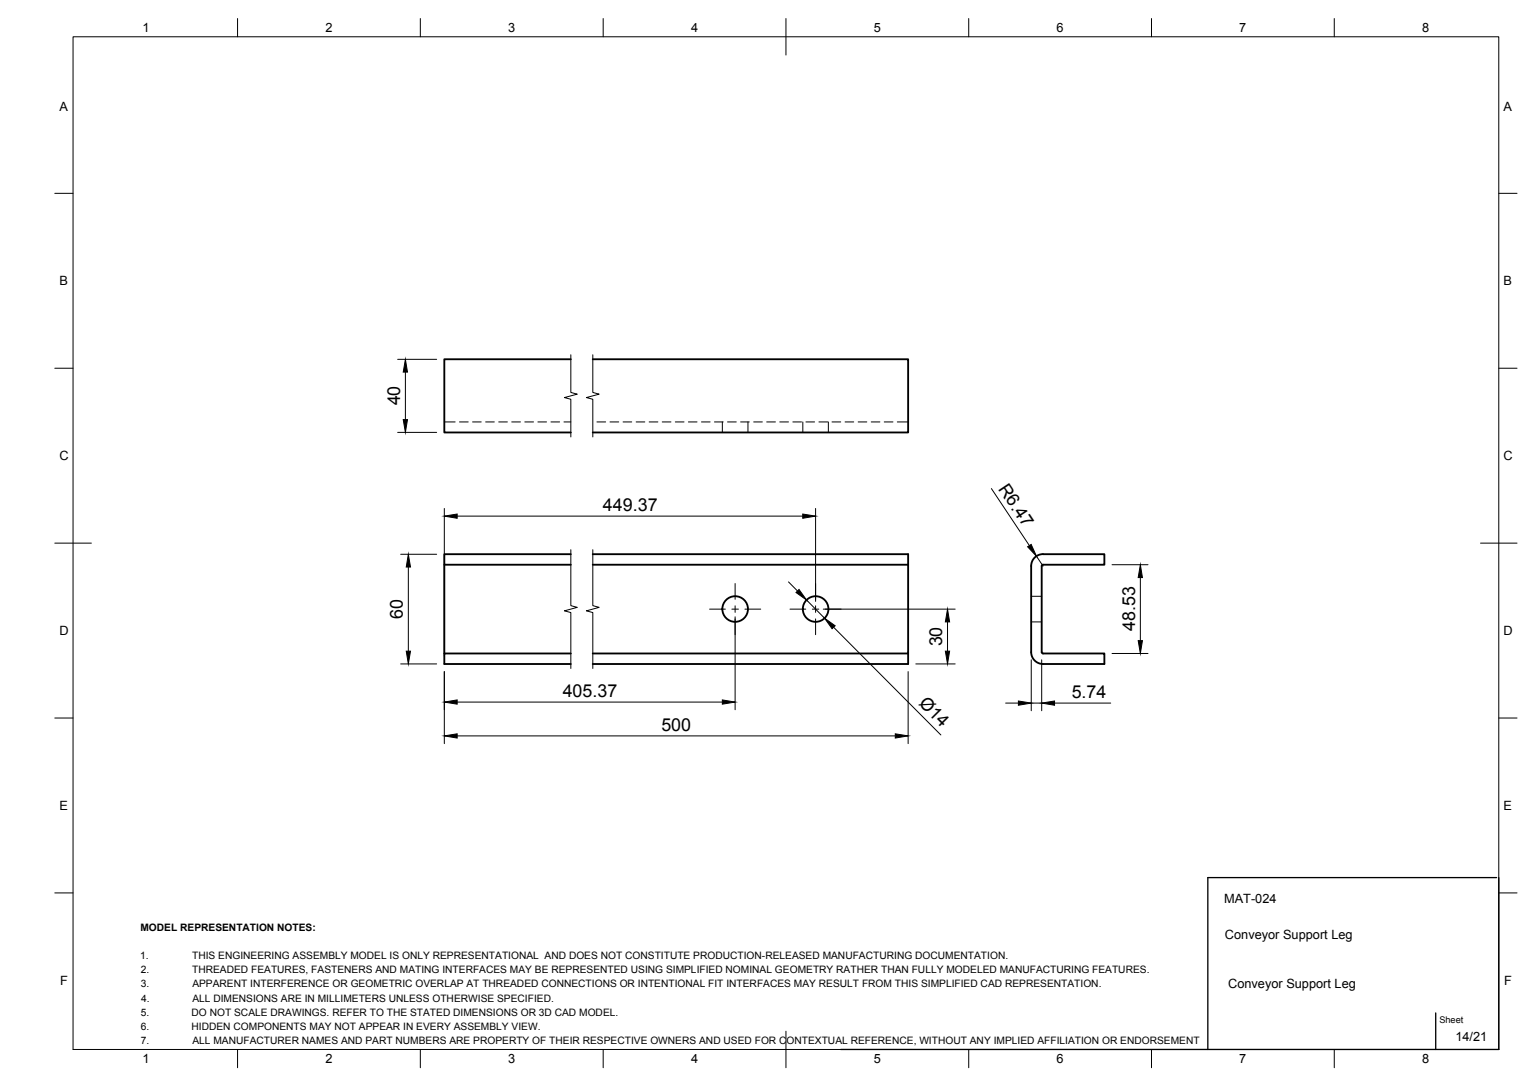
ISO-10303-21;
HEADER;
/* Generated by software containing ST-Developer
 * from STEP Tools, Inc. (www.steptools.com) 
 */

FILE_DESCRIPTION(
/* description */ ('STEP AP214'),
/* implementation_level */ '2;1');

FILE_NAME(
/* name */ 'Conveyor Support Leg.step',
/* time_stamp */ '2026-11-14T06:34:07-08:00',
/* author */ (''),
/* organization */ (''),
/* preprocessor_version */ 'ST-DEVELOPER v20.2',
/* originating_system */ 'Autodesk Translation Framework v15.17.0.0',
/* authorisation */ '');

FILE_SCHEMA (('AUTOMOTIVE_DESIGN { 1 0 10303 214 3 1 1 }'));
ENDSEC;

DATA;
#10=MECHANICAL_DESIGN_GEOMETRIC_PRESENTATION_REPRESENTATION('',(#7321),#310623);
#7236=SHAPE_REPRESENTATION_RELATIONSHIP('SRR','None',#310910,#7253);
#7253=ADVANCED_BREP_SHAPE_REPRESENTATION('',(#7388),#310619);
#7321=STYLED_ITEM('',(#311003),#7388);
#7388=MANIFOLD_SOLID_BREP('Body1',#93772);
#7692=FACE_BOUND('',#20319,.T.);
#7693=FACE_BOUND('',#20320,.T.);
#7694=FACE_BOUND('',#20324,.T.);
#7695=FACE_BOUND('',#20325,.T.);
#8642=PLANE('',#104604);
#8643=PLANE('',#104605);
#8644=PLANE('',#104606);
#8645=PLANE('',#104607);
#8646=PLANE('',#104608);
#8647=PLANE('',#104609);
#8648=PLANE('',#104610);
#8649=PLANE('',#104611);
#8650=PLANE('',#104612);
#8651=PLANE('',#104615);
#8652=PLANE('',#104616);
#8653=PLANE('',#104619);
#8654=PLANE('',#104622);
#8655=PLANE('',#104625);
#8656=PLANE('',#104627);
#8657=PLANE('',#104630);
#8658=PLANE('',#104632);
#8659=PLANE('',#104633);
#14261=FACE_OUTER_BOUND('',#20301,.T.);
#14262=FACE_OUTER_BOUND('',#20302,.T.);
#14263=FACE_OUTER_BOUND('',#20303,.T.);
#14264=FACE_OUTER_BOUND('',#20304,.T.);
#14265=FACE_OUTER_BOUND('',#20305,.T.);
#14266=FACE_OUTER_BOUND('',#20306,.T.);
#14267=FACE_OUTER_BOUND('',#20307,.T.);
#14268=FACE_OUTER_BOUND('',#20308,.T.);
#14269=FACE_OUTER_BOUND('',#20309,.T.);
#14270=FACE_OUTER_BOUND('',#20310,.T.);
#14271=FACE_OUTER_BOUND('',#20311,.T.);
#14272=FACE_OUTER_BOUND('',#20312,.T.);
#14273=FACE_OUTER_BOUND('',#20313,.T.);
#14274=FACE_OUTER_BOUND('',#20314,.T.);
#14275=FACE_OUTER_BOUND('',#20315,.T.);
#14276=FACE_OUTER_BOUND('',#20316,.T.);
#14277=FACE_OUTER_BOUND('',#20317,.T.);
#14278=FACE_OUTER_BOUND('',#20318,.T.);
#14279=FACE_OUTER_BOUND('',#20321,.T.);
#14280=FACE_OUTER_BOUND('',#20322,.T.);
#14281=FACE_OUTER_BOUND('',#20323,.T.);
#14282=FACE_OUTER_BOUND('',#20326,.T.);
#14283=FACE_OUTER_BOUND('',#20327,.T.);
#14284=FACE_OUTER_BOUND('',#20328,.T.);
#20301=EDGE_LOOP('',(#84911,#84912,#84913,#84914));
#20302=EDGE_LOOP('',(#84915,#84916,#84917,#84918));
#20303=EDGE_LOOP('',(#84919,#84920,#84921,#84922));
#20304=EDGE_LOOP('',(#84923,#84924,#84925,#84926));
#20305=EDGE_LOOP('',(#84927,#84928,#84929,#84930));
#20306=EDGE_LOOP('',(#84931,#84932,#84933,#84934));
#20307=EDGE_LOOP('',(#84935,#84936,#84937,#84938));
#20308=EDGE_LOOP('',(#84939,#84940,#84941,#84942));
#20309=EDGE_LOOP('',(#84943,#84944,#84945,#84946));
#20310=EDGE_LOOP('',(#84947,#84948,#84949,#84950));
#20311=EDGE_LOOP('',(#84951,#84952,#84953,#84954));
#20312=EDGE_LOOP('',(#84955,#84956,#84957,#84958));
#20313=EDGE_LOOP('',(#84959,#84960,#84961,#84962));
#20314=EDGE_LOOP('',(#84963,#84964,#84965,#84966));
#20315=EDGE_LOOP('',(#84967,#84968,#84969,#84970));
#20316=EDGE_LOOP('',(#84971,#84972,#84973,#84974));
#20317=EDGE_LOOP('',(#84975,#84976,#84977,#84978));
#20318=EDGE_LOOP('',(#84979,#84980,#84981,#84982));
#20319=EDGE_LOOP('',(#84983));
#20320=EDGE_LOOP('',(#84984));
#20321=EDGE_LOOP('',(#84985,#84986,#84987,#84988));
#20322=EDGE_LOOP('',(#84989,#84990,#84991,#84992));
#20323=EDGE_LOOP('',(#84993,#84994,#84995,#84996));
#20324=EDGE_LOOP('',(#84997));
#20325=EDGE_LOOP('',(#84998));
#20326=EDGE_LOOP('',(#84999,#85000,#85001,#85002));
#20327=EDGE_LOOP('',(#85003,#85004,#85005,#85006));
#20328=EDGE_LOOP('',(#85007,#85008,#85009,#85010));
#24672=LINE('',#302915,#29019);
#24673=LINE('',#302921,#29020);
#24674=LINE('',#302926,#29021);
#24675=LINE('',#302928,#29022);
#24676=LINE('',#302930,#29023);
#24677=LINE('',#302931,#29024);
#24678=LINE('',#302935,#29025);
#24679=LINE('',#302937,#29026);
#24680=LINE('',#302939,#29027);
#24681=LINE('',#302940,#29028);
#24682=LINE('',#302943,#29029);
#24683=LINE('',#302945,#29030);
#24684=LINE('',#302946,#29031);
#24685=LINE('',#302949,#29032);
#24686=LINE('',#302951,#29033);
#24687=LINE('',#302952,#29034);
#24688=LINE('',#302955,#29035);
#24689=LINE('',#302957,#29036);
#24690=LINE('',#302958,#29037);
#24691=LINE('',#302961,#29038);
#24692=LINE('',#302963,#29039);
#24693=LINE('',#302964,#29040);
#24694=LINE('',#302966,#29041);
#24695=LINE('',#302967,#29042);
#24696=LINE('',#302969,#29043);
#24697=LINE('',#302970,#29044);
#24698=LINE('',#302974,#29045);
#24699=LINE('',#302979,#29046);
#24700=LINE('',#302981,#29047);
#24701=LINE('',#302982,#29048);
#24702=LINE('',#302987,#29049);
#24703=LINE('',#302995,#29050);
#24704=LINE('',#302999,#29051);
#24705=LINE('',#303000,#29052);
#24706=LINE('',#303002,#29053);
#24707=LINE('',#303004,#29054);
#24708=LINE('',#303007,#29055);
#24709=LINE('',#303009,#29056);
#29019=VECTOR('',#130329,7.00000000000001);
#29020=VECTOR('',#130336,7.);
#29021=VECTOR('',#130341,1000.);
#29022=VECTOR('',#130342,1000.);
#29023=VECTOR('',#130343,1000.);
#29024=VECTOR('',#130344,1000.);
#29025=VECTOR('',#130347,1000.);
#29026=VECTOR('',#130348,1000.);
#29027=VECTOR('',#130349,1000.);
#29028=VECTOR('',#130350,1000.);
#29029=VECTOR('',#130353,1000.);
#29030=VECTOR('',#130354,1000.);
#29031=VECTOR('',#130355,1000.);
#29032=VECTOR('',#130358,1000.);
#29033=VECTOR('',#130359,1000.);
#29034=VECTOR('',#130360,1000.);
#29035=VECTOR('',#130363,1000.);
#29036=VECTOR('',#130364,1000.);
#29037=VECTOR('',#130365,1000.);
#29038=VECTOR('',#130368,1000.);
#29039=VECTOR('',#130369,1000.);
#29040=VECTOR('',#130370,1000.);
#29041=VECTOR('',#130373,1000.);
#29042=VECTOR('',#130374,1000.);
#29043=VECTOR('',#130377,1000.);
#29044=VECTOR('',#130378,1000.);
#29045=VECTOR('',#130381,1000.);
#29046=VECTOR('',#130388,1000.);
#29047=VECTOR('',#130389,1000.);
#29048=VECTOR('',#130390,1000.);
#29049=VECTOR('',#130395,1000.);
#29050=VECTOR('',#130406,1000.);
#29051=VECTOR('',#130413,1000.);
#29052=VECTOR('',#130414,1000.);
#29053=VECTOR('',#130417,1000.);
#29054=VECTOR('',#130420,1000.);
#29055=VECTOR('',#130425,1000.);
#29056=VECTOR('',#130428,1000.);
#35057=CIRCLE('',#104599,7.00000000000001);
#35058=CIRCLE('',#104600,7.00000000000001);
#35059=CIRCLE('',#104602,7.);
#35060=CIRCLE('',#104603,7.);
#35061=CIRCLE('',#104613,6.4732);
#35062=CIRCLE('',#104614,0.736599999999997);
#35063=CIRCLE('',#104617,6.4732);
#35064=CIRCLE('',#104618,0.736599999999997);
#35065=CIRCLE('',#104620,6.4732);
#35066=CIRCLE('',#104621,0.736599999999997);
#35067=CIRCLE('',#104623,6.4732);
#35068=CIRCLE('',#104624,0.736599999999997);
#43338=VERTEX_POINT('',#302912);
#43339=VERTEX_POINT('',#302914);
#43340=VERTEX_POINT('',#302918);
#43341=VERTEX_POINT('',#302920);
#43342=VERTEX_POINT('',#302924);
#43343=VERTEX_POINT('',#302925);
#43344=VERTEX_POINT('',#302927);
#43345=VERTEX_POINT('',#302929);
#43346=VERTEX_POINT('',#302933);
#43347=VERTEX_POINT('',#302934);
#43348=VERTEX_POINT('',#302936);
#43349=VERTEX_POINT('',#302938);
#43350=VERTEX_POINT('',#302942);
#43351=VERTEX_POINT('',#302944);
#43352=VERTEX_POINT('',#302948);
#43353=VERTEX_POINT('',#302950);
#43354=VERTEX_POINT('',#302954);
#43355=VERTEX_POINT('',#302956);
#43356=VERTEX_POINT('',#302960);
#43357=VERTEX_POINT('',#302962);
#43358=VERTEX_POINT('',#302972);
#43359=VERTEX_POINT('',#302973);
#43360=VERTEX_POINT('',#302978);
#43361=VERTEX_POINT('',#302980);
#43362=VERTEX_POINT('',#302984);
#43363=VERTEX_POINT('',#302986);
#43364=VERTEX_POINT('',#302993);
#43365=VERTEX_POINT('',#302994);
#57235=EDGE_CURVE('',#43338,#43338,#35057,.T.);
#57236=EDGE_CURVE('',#43338,#43339,#24672,.T.);
#57237=EDGE_CURVE('',#43339,#43339,#35058,.T.);
#57238=EDGE_CURVE('',#43340,#43340,#35059,.T.);
#57239=EDGE_CURVE('',#43340,#43341,#24673,.T.);
#57240=EDGE_CURVE('',#43341,#43341,#35060,.T.);
#57241=EDGE_CURVE('',#43342,#43343,#24674,.T.);
#57242=EDGE_CURVE('',#43342,#43344,#24675,.T.);
#57243=EDGE_CURVE('',#43344,#43345,#24676,.T.);
#57244=EDGE_CURVE('',#43345,#43343,#24677,.T.);
#57245=EDGE_CURVE('',#43346,#43347,#24678,.T.);
#57246=EDGE_CURVE('',#43347,#43348,#24679,.T.);
#57247=EDGE_CURVE('',#43349,#43348,#24680,.T.);
#57248=EDGE_CURVE('',#43349,#43346,#24681,.T.);
#57249=EDGE_CURVE('',#43347,#43350,#24682,.T.);
#57250=EDGE_CURVE('',#43346,#43351,#24683,.T.);
#57251=EDGE_CURVE('',#43351,#43350,#24684,.T.);
#57252=EDGE_CURVE('',#43348,#43352,#24685,.T.);
#57253=EDGE_CURVE('',#43353,#43352,#24686,.T.);
#57254=EDGE_CURVE('',#43349,#43353,#24687,.T.);
#57255=EDGE_CURVE('',#43344,#43354,#24688,.T.);
#57256=EDGE_CURVE('',#43354,#43355,#24689,.T.);
#57257=EDGE_CURVE('',#43355,#43345,#24690,.T.);
#57258=EDGE_CURVE('',#43342,#43356,#24691,.T.);
#57259=EDGE_CURVE('',#43357,#43343,#24692,.T.);
#57260=EDGE_CURVE('',#43356,#43357,#24693,.T.);
#57261=EDGE_CURVE('',#43354,#43356,#24694,.T.);
#57262=EDGE_CURVE('',#43357,#43355,#24695,.T.);
#57263=EDGE_CURVE('',#43350,#43352,#24696,.T.);
#57264=EDGE_CURVE('',#43351,#43353,#24697,.T.);
#57265=EDGE_CURVE('',#43358,#43359,#24698,.T.);
#57266=EDGE_CURVE('',#43355,#43358,#35061,.T.);
#57267=EDGE_CURVE('',#43357,#43359,#35062,.T.);
#57268=EDGE_CURVE('',#43358,#43360,#24699,.T.);
#57269=EDGE_CURVE('',#43359,#43361,#24700,.T.);
#57270=EDGE_CURVE('',#43361,#43360,#24701,.T.);
#57271=EDGE_CURVE('',#43345,#43362,#35063,.T.);
#57272=EDGE_CURVE('',#43363,#43362,#24702,.T.);
#57273=EDGE_CURVE('',#43343,#43363,#35064,.T.);
#57274=EDGE_CURVE('',#43360,#43349,#35065,.T.);
#57275=EDGE_CURVE('',#43361,#43346,#35066,.T.);
#57276=EDGE_CURVE('',#43364,#43365,#24703,.T.);
#57277=EDGE_CURVE('',#43364,#43353,#35067,.T.);
#57278=EDGE_CURVE('',#43365,#43351,#35068,.T.);
#57279=EDGE_CURVE('',#43362,#43364,#24704,.T.);
#57280=EDGE_CURVE('',#43363,#43365,#24705,.T.);
#57281=EDGE_CURVE('',#43360,#43364,#24706,.T.);
#57282=EDGE_CURVE('',#43358,#43362,#24707,.T.);
#57283=EDGE_CURVE('',#43359,#43363,#24708,.T.);
#57284=EDGE_CURVE('',#43361,#43365,#24709,.T.);
#84911=ORIENTED_EDGE('',*,*,#57235,.F.);
#84912=ORIENTED_EDGE('',*,*,#57236,.T.);
#84913=ORIENTED_EDGE('',*,*,#57237,.T.);
#84914=ORIENTED_EDGE('',*,*,#57236,.F.);
#84915=ORIENTED_EDGE('',*,*,#57238,.F.);
#84916=ORIENTED_EDGE('',*,*,#57239,.T.);
#84917=ORIENTED_EDGE('',*,*,#57240,.T.);
#84918=ORIENTED_EDGE('',*,*,#57239,.F.);
#84919=ORIENTED_EDGE('',*,*,#57241,.F.);
#84920=ORIENTED_EDGE('',*,*,#57242,.T.);
#84921=ORIENTED_EDGE('',*,*,#57243,.T.);
#84922=ORIENTED_EDGE('',*,*,#57244,.T.);
#84923=ORIENTED_EDGE('',*,*,#57245,.T.);
#84924=ORIENTED_EDGE('',*,*,#57246,.T.);
#84925=ORIENTED_EDGE('',*,*,#57247,.F.);
#84926=ORIENTED_EDGE('',*,*,#57248,.T.);
#84927=ORIENTED_EDGE('',*,*,#57249,.F.);
#84928=ORIENTED_EDGE('',*,*,#57245,.F.);
#84929=ORIENTED_EDGE('',*,*,#57250,.T.);
#84930=ORIENTED_EDGE('',*,*,#57251,.T.);
#84931=ORIENTED_EDGE('',*,*,#57247,.T.);
#84932=ORIENTED_EDGE('',*,*,#57252,.T.);
#84933=ORIENTED_EDGE('',*,*,#57253,.F.);
#84934=ORIENTED_EDGE('',*,*,#57254,.F.);
#84935=ORIENTED_EDGE('',*,*,#57243,.F.);
#84936=ORIENTED_EDGE('',*,*,#57255,.T.);
#84937=ORIENTED_EDGE('',*,*,#57256,.T.);
#84938=ORIENTED_EDGE('',*,*,#57257,.T.);
#84939=ORIENTED_EDGE('',*,*,#57258,.F.);
#84940=ORIENTED_EDGE('',*,*,#57241,.T.);
#84941=ORIENTED_EDGE('',*,*,#57259,.F.);
#84942=ORIENTED_EDGE('',*,*,#57260,.F.);
#84943=ORIENTED_EDGE('',*,*,#57256,.F.);
#84944=ORIENTED_EDGE('',*,*,#57261,.T.);
#84945=ORIENTED_EDGE('',*,*,#57260,.T.);
#84946=ORIENTED_EDGE('',*,*,#57262,.T.);
#84947=ORIENTED_EDGE('',*,*,#57263,.F.);
#84948=ORIENTED_EDGE('',*,*,#57251,.F.);
#84949=ORIENTED_EDGE('',*,*,#57264,.T.);
#84950=ORIENTED_EDGE('',*,*,#57253,.T.);
#84951=ORIENTED_EDGE('',*,*,#57265,.F.);
#84952=ORIENTED_EDGE('',*,*,#57266,.F.);
#84953=ORIENTED_EDGE('',*,*,#57262,.F.);
#84954=ORIENTED_EDGE('',*,*,#57267,.T.);
#84955=ORIENTED_EDGE('',*,*,#57268,.F.);
#84956=ORIENTED_EDGE('',*,*,#57265,.T.);
#84957=ORIENTED_EDGE('',*,*,#57269,.T.);
#84958=ORIENTED_EDGE('',*,*,#57270,.T.);
#84959=ORIENTED_EDGE('',*,*,#57244,.F.);
#84960=ORIENTED_EDGE('',*,*,#57271,.T.);
#84961=ORIENTED_EDGE('',*,*,#57272,.F.);
#84962=ORIENTED_EDGE('',*,*,#57273,.F.);
#84963=ORIENTED_EDGE('',*,*,#57248,.F.);
#84964=ORIENTED_EDGE('',*,*,#57274,.F.);
#84965=ORIENTED_EDGE('',*,*,#57270,.F.);
#84966=ORIENTED_EDGE('',*,*,#57275,.T.);
#84967=ORIENTED_EDGE('',*,*,#57276,.F.);
#84968=ORIENTED_EDGE('',*,*,#57277,.T.);
#84969=ORIENTED_EDGE('',*,*,#57264,.F.);
#84970=ORIENTED_EDGE('',*,*,#57278,.F.);
#84971=ORIENTED_EDGE('',*,*,#57279,.T.);
#84972=ORIENTED_EDGE('',*,*,#57276,.T.);
#84973=ORIENTED_EDGE('',*,*,#57280,.F.);
#84974=ORIENTED_EDGE('',*,*,#57272,.T.);
#84975=ORIENTED_EDGE('',*,*,#57277,.F.);
#84976=ORIENTED_EDGE('',*,*,#57281,.F.);
#84977=ORIENTED_EDGE('',*,*,#57274,.T.);
#84978=ORIENTED_EDGE('',*,*,#57254,.T.);
#84979=ORIENTED_EDGE('',*,*,#57279,.F.);
#84980=ORIENTED_EDGE('',*,*,#57282,.F.);
#84981=ORIENTED_EDGE('',*,*,#57268,.T.);
#84982=ORIENTED_EDGE('',*,*,#57281,.T.);
#84983=ORIENTED_EDGE('',*,*,#57237,.F.);
#84984=ORIENTED_EDGE('',*,*,#57240,.F.);
#84985=ORIENTED_EDGE('',*,*,#57271,.F.);
#84986=ORIENTED_EDGE('',*,*,#57257,.F.);
#84987=ORIENTED_EDGE('',*,*,#57266,.T.);
#84988=ORIENTED_EDGE('',*,*,#57282,.T.);
#84989=ORIENTED_EDGE('',*,*,#57273,.T.);
#84990=ORIENTED_EDGE('',*,*,#57283,.F.);
#84991=ORIENTED_EDGE('',*,*,#57267,.F.);
#84992=ORIENTED_EDGE('',*,*,#57259,.T.);
#84993=ORIENTED_EDGE('',*,*,#57280,.T.);
#84994=ORIENTED_EDGE('',*,*,#57284,.F.);
#84995=ORIENTED_EDGE('',*,*,#57269,.F.);
#84996=ORIENTED_EDGE('',*,*,#57283,.T.);
#84997=ORIENTED_EDGE('',*,*,#57235,.T.);
#84998=ORIENTED_EDGE('',*,*,#57238,.T.);
#84999=ORIENTED_EDGE('',*,*,#57278,.T.);
#85000=ORIENTED_EDGE('',*,*,#57250,.F.);
#85001=ORIENTED_EDGE('',*,*,#57275,.F.);
#85002=ORIENTED_EDGE('',*,*,#57284,.T.);
#85003=ORIENTED_EDGE('',*,*,#57249,.T.);
#85004=ORIENTED_EDGE('',*,*,#57263,.T.);
#85005=ORIENTED_EDGE('',*,*,#57252,.F.);
#85006=ORIENTED_EDGE('',*,*,#57246,.F.);
#85007=ORIENTED_EDGE('',*,*,#57258,.T.);
#85008=ORIENTED_EDGE('',*,*,#57261,.F.);
#85009=ORIENTED_EDGE('',*,*,#57255,.F.);
#85010=ORIENTED_EDGE('',*,*,#57242,.F.);
#87908=CYLINDRICAL_SURFACE('',#104598,7.00000000000001);
#87909=CYLINDRICAL_SURFACE('',#104601,7.);
#87910=CYLINDRICAL_SURFACE('',#104626,6.4732);
#87911=CYLINDRICAL_SURFACE('',#104628,6.4732);
#87912=CYLINDRICAL_SURFACE('',#104629,0.7366);
#87913=CYLINDRICAL_SURFACE('',#104631,0.736599999999997);
#93540=ADVANCED_FACE('',(#14261),#87908,.F.);
#93541=ADVANCED_FACE('',(#14262),#87909,.F.);
#93542=ADVANCED_FACE('',(#14263),#8642,.T.);
#93543=ADVANCED_FACE('',(#14264),#8643,.T.);
#93544=ADVANCED_FACE('',(#14265),#8644,.F.);
#93545=ADVANCED_FACE('',(#14266),#8645,.T.);
#93546=ADVANCED_FACE('',(#14267),#8646,.T.);
#93547=ADVANCED_FACE('',(#14268),#8647,.F.);
#93548=ADVANCED_FACE('',(#14269),#8648,.T.);
#93549=ADVANCED_FACE('',(#14270),#8649,.F.);
#93550=ADVANCED_FACE('',(#14271),#8650,.T.);
#93551=ADVANCED_FACE('',(#14272),#8651,.T.);
#93552=ADVANCED_FACE('',(#14273),#8652,.T.);
#93553=ADVANCED_FACE('',(#14274),#8653,.T.);
#93554=ADVANCED_FACE('',(#14275),#8654,.T.);
#93555=ADVANCED_FACE('',(#14276),#8655,.T.);
#93556=ADVANCED_FACE('',(#14277),#87910,.T.);
#93557=ADVANCED_FACE('',(#14278,#7692,#7693),#8656,.T.);
#93558=ADVANCED_FACE('',(#14279),#87911,.T.);
#93559=ADVANCED_FACE('',(#14280),#87912,.F.);
#93560=ADVANCED_FACE('',(#14281,#7694,#7695),#8657,.F.);
#93561=ADVANCED_FACE('',(#14282),#87913,.F.);
#93562=ADVANCED_FACE('',(#14283),#8658,.T.);
#93563=ADVANCED_FACE('',(#14284),#8659,.T.);
#93772=CLOSED_SHELL('',(#93540,#93541,#93542,#93543,#93544,#93545,#93546,
#93547,#93548,#93549,#93550,#93551,#93552,#93553,#93554,#93555,#93556,#93557,
#93558,#93559,#93560,#93561,#93562,#93563));
#104597=AXIS2_PLACEMENT_3D('',#302910,#130323,#130324);
#104598=AXIS2_PLACEMENT_3D('',#302911,#130325,#130326);
#104599=AXIS2_PLACEMENT_3D('',#302913,#130327,#130328);
#104600=AXIS2_PLACEMENT_3D('',#302916,#130330,#130331);
#104601=AXIS2_PLACEMENT_3D('',#302917,#130332,#130333);
#104602=AXIS2_PLACEMENT_3D('',#302919,#130334,#130335);
#104603=AXIS2_PLACEMENT_3D('',#302922,#130337,#130338);
#104604=AXIS2_PLACEMENT_3D('',#302923,#130339,#130340);
#104605=AXIS2_PLACEMENT_3D('',#302932,#130345,#130346);
#104606=AXIS2_PLACEMENT_3D('',#302941,#130351,#130352);
#104607=AXIS2_PLACEMENT_3D('',#302947,#130356,#130357);
#104608=AXIS2_PLACEMENT_3D('',#302953,#130361,#130362);
#104609=AXIS2_PLACEMENT_3D('',#302959,#130366,#130367);
#104610=AXIS2_PLACEMENT_3D('',#302965,#130371,#130372);
#104611=AXIS2_PLACEMENT_3D('',#302968,#130375,#130376);
#104612=AXIS2_PLACEMENT_3D('',#302971,#130379,#130380);
#104613=AXIS2_PLACEMENT_3D('',#302975,#130382,#130383);
#104614=AXIS2_PLACEMENT_3D('',#302976,#130384,#130385);
#104615=AXIS2_PLACEMENT_3D('',#302977,#130386,#130387);
#104616=AXIS2_PLACEMENT_3D('',#302983,#130391,#130392);
#104617=AXIS2_PLACEMENT_3D('',#302985,#130393,#130394);
#104618=AXIS2_PLACEMENT_3D('',#302988,#130396,#130397);
#104619=AXIS2_PLACEMENT_3D('',#302989,#130398,#130399);
#104620=AXIS2_PLACEMENT_3D('',#302990,#130400,#130401);
#104621=AXIS2_PLACEMENT_3D('',#302991,#130402,#130403);
#104622=AXIS2_PLACEMENT_3D('',#302992,#130404,#130405);
#104623=AXIS2_PLACEMENT_3D('',#302996,#130407,#130408);
#104624=AXIS2_PLACEMENT_3D('',#302997,#130409,#130410);
#104625=AXIS2_PLACEMENT_3D('',#302998,#130411,#130412);
#104626=AXIS2_PLACEMENT_3D('',#303001,#130415,#130416);
#104627=AXIS2_PLACEMENT_3D('',#303003,#130418,#130419);
#104628=AXIS2_PLACEMENT_3D('',#303005,#130421,#130422);
#104629=AXIS2_PLACEMENT_3D('',#303006,#130423,#130424);
#104630=AXIS2_PLACEMENT_3D('',#303008,#130426,#130427);
#104631=AXIS2_PLACEMENT_3D('',#303010,#130429,#130430);
#104632=AXIS2_PLACEMENT_3D('',#303011,#130431,#130432);
#104633=AXIS2_PLACEMENT_3D('',#303012,#130433,#130434);
#130323=DIRECTION('axis',(0.,0.,1.));
#130324=DIRECTION('refdir',(1.,0.,0.));
#130325=DIRECTION('center_axis',(-1.,7.59645419660784E-65,0.));
#130326=DIRECTION('ref_axis',(0.,0.,1.));
#130327=DIRECTION('center_axis',(-1.,7.59645419660784E-65,0.));
#130328=DIRECTION('ref_axis',(0.,0.,1.));
#130329=DIRECTION('',(-1.,7.59645419660784E-65,0.));
#130330=DIRECTION('center_axis',(-1.,7.59645419660784E-65,0.));
#130331=DIRECTION('ref_axis',(0.,0.,1.));
#130332=DIRECTION('center_axis',(-1.,7.59645419660784E-65,0.));
#130333=DIRECTION('ref_axis',(0.,0.,1.));
#130334=DIRECTION('center_axis',(-1.,7.59645419660784E-65,0.));
#130335=DIRECTION('ref_axis',(0.,0.,1.));
#130336=DIRECTION('',(-1.,7.59645419660784E-65,0.));
#130337=DIRECTION('center_axis',(-1.,7.59645419660784E-65,0.));
#130338=DIRECTION('ref_axis',(0.,0.,1.));
#130339=DIRECTION('center_axis',(7.59645419660784E-65,-1.,0.));
#130340=DIRECTION('ref_axis',(0.,0.,-1.));
#130341=DIRECTION('',(-1.,0.,1.22464679914735E-16));
#130342=DIRECTION('',(0.,0.,1.));
#130343=DIRECTION('',(-1.,0.,1.22464679914735E-16));
#130344=DIRECTION('',(0.,0.,-1.));
#130345=DIRECTION('center_axis',(-7.59645419660784E-65,1.,0.));
#130346=DIRECTION('ref_axis',(0.,0.,1.));
#130347=DIRECTION('',(1.,-7.59645419660784E-65,0.));
#130348=DIRECTION('',(0.,0.,-1.));
#130349=DIRECTION('',(1.,-7.59645419660784E-65,0.));
#130350=DIRECTION('',(0.,0.,1.));
#130351=DIRECTION('center_axis',(0.,0.,-1.));
#130352=DIRECTION('ref_axis',(-1.,7.59645419660784E-65,0.));
#130353=DIRECTION('',(7.59645419660784E-65,-1.,0.));
#130354=DIRECTION('',(7.59645419660784E-65,-1.,0.));
#130355=DIRECTION('',(1.,-7.59645419660784E-65,0.));
#130356=DIRECTION('center_axis',(0.,0.,-1.));
#130357=DIRECTION('ref_axis',(-1.,7.59645419660784E-65,0.));
#130358=DIRECTION('',(7.59645419660784E-65,-1.,0.));
#130359=DIRECTION('',(1.,-7.59645419660784E-65,0.));
#130360=DIRECTION('',(7.59645419660784E-65,-1.,0.));
#130361=DIRECTION('center_axis',(1.22464679914735E-16,0.,1.));
#130362=DIRECTION('ref_axis',(1.,0.,-1.22464679914735E-16));
#130363=DIRECTION('',(-7.59645419660784E-65,1.,0.));
#130364=DIRECTION('',(-1.,0.,1.22464679914735E-16));
#130365=DIRECTION('',(7.59645419660784E-65,-1.,0.));
#130366=DIRECTION('center_axis',(1.22464679914735E-16,0.,1.));
#130367=DIRECTION('ref_axis',(1.,0.,-1.22464679914735E-16));
#130368=DIRECTION('',(-7.59645419660784E-65,1.,0.));
#130369=DIRECTION('',(7.59645419660784E-65,-1.,0.));
#130370=DIRECTION('',(-1.,0.,1.22464679914735E-16));
#130371=DIRECTION('center_axis',(7.59645419660784E-65,1.,0.));
#130372=DIRECTION('ref_axis',(1.,-7.59645419660784E-65,0.));
#130373=DIRECTION('',(0.,0.,-1.));
#130374=DIRECTION('',(0.,0.,1.));
#130375=DIRECTION('center_axis',(7.59645419660784E-65,1.,0.));
#130376=DIRECTION('ref_axis',(1.,-7.59645419660784E-65,0.));
#130377=DIRECTION('',(0.,0.,-1.));
#130378=DIRECTION('',(0.,0.,-1.));
#130379=DIRECTION('center_axis',(-7.59645419660784E-65,1.,0.));
#130380=DIRECTION('ref_axis',(0.,0.,1.));
#130381=DIRECTION('',(1.,-7.59645419660784E-65,0.));
#130382=DIRECTION('center_axis',(7.59645419660784E-65,-1.,0.));
#130383=DIRECTION('ref_axis',(0.,0.,1.));
#130384=DIRECTION('center_axis',(7.59645419660784E-65,-1.,0.));
#130385=DIRECTION('ref_axis',(1.,7.59645419660784E-65,0.));
#130386=DIRECTION('center_axis',(-7.59645419660784E-65,1.,0.));
#130387=DIRECTION('ref_axis',(0.,0.,1.));
#130388=DIRECTION('',(0.,0.,-1.));
#130389=DIRECTION('',(0.,0.,-1.));
#130390=DIRECTION('',(-1.,7.59645419660784E-65,0.));
#130391=DIRECTION('center_axis',(7.59645419660784E-65,-1.,0.));
#130392=DIRECTION('ref_axis',(0.,0.,-1.));
#130393=DIRECTION('center_axis',(7.59645419660784E-65,-1.,0.));
#130394=DIRECTION('ref_axis',(0.,0.,1.));
#130395=DIRECTION('',(-1.,7.59645419660784E-65,0.));
#130396=DIRECTION('center_axis',(7.59645419660784E-65,-1.,0.));
#130397=DIRECTION('ref_axis',(1.,7.59645419660784E-65,0.));
#130398=DIRECTION('center_axis',(-7.59645419660784E-65,1.,0.));
#130399=DIRECTION('ref_axis',(0.,0.,1.));
#130400=DIRECTION('center_axis',(7.59645419660784E-65,-1.,0.));
#130401=DIRECTION('ref_axis',(0.,0.,1.));
#130402=DIRECTION('center_axis',(7.59645419660784E-65,-1.,0.));
#130403=DIRECTION('ref_axis',(1.,7.59645419660784E-65,0.));
#130404=DIRECTION('center_axis',(7.59645419660784E-65,-1.,0.));
#130405=DIRECTION('ref_axis',(0.,0.,-1.));
#130406=DIRECTION('',(1.,-7.59645419660784E-65,0.));
#130407=DIRECTION('center_axis',(7.59645419660784E-65,-1.,0.));
#130408=DIRECTION('ref_axis',(0.,0.,1.));
#130409=DIRECTION('center_axis',(7.59645419660784E-65,-1.,0.));
#130410=DIRECTION('ref_axis',(1.,7.59645419660784E-65,0.));
#130411=DIRECTION('center_axis',(7.59645419660784E-65,-1.,0.));
#130412=DIRECTION('ref_axis',(0.,0.,-1.));
#130413=DIRECTION('',(0.,0.,-1.));
#130414=DIRECTION('',(0.,0.,-1.));
#130415=DIRECTION('center_axis',(7.59645419660784E-65,-1.,0.));
#130416=DIRECTION('ref_axis',(0.,0.,-1.));
#130417=DIRECTION('',(7.59645419660784E-65,-1.,0.));
#130418=DIRECTION('center_axis',(-1.,7.59645419660784E-65,0.));
#130419=DIRECTION('ref_axis',(0.,0.,1.));
#130420=DIRECTION('',(7.59645419660784E-65,-1.,0.));
#130421=DIRECTION('center_axis',(7.59645419660784E-65,-1.,0.));
#130422=DIRECTION('ref_axis',(0.,0.,-1.));
#130423=DIRECTION('center_axis',(7.59645419660784E-65,-1.,0.));
#130424=DIRECTION('ref_axis',(0.,0.,-1.));
#130425=DIRECTION('',(7.59645419660784E-65,-1.,0.));
#130426=DIRECTION('center_axis',(-1.,7.59645419660784E-65,0.));
#130427=DIRECTION('ref_axis',(0.,0.,1.));
#130428=DIRECTION('',(7.59645419660784E-65,-1.,0.));
#130429=DIRECTION('center_axis',(7.59645419660784E-65,-1.,0.));
#130430=DIRECTION('ref_axis',(0.,0.,-1.));
#130431=DIRECTION('center_axis',(1.,-7.59645419660784E-65,0.));
#130432=DIRECTION('ref_axis',(0.,0.,-1.));
#130433=DIRECTION('center_axis',(1.,-7.59645419660784E-65,0.));
#130434=DIRECTION('ref_axis',(0.,0.,-1.));
#302910=CARTESIAN_POINT('',(0.,0.,0.));
#302911=CARTESIAN_POINT('Origin',(0.,94.6262929075966,-30.));
#302912=CARTESIAN_POINT('',(-44.2634,94.6262929075966,-37.));
#302913=CARTESIAN_POINT('Origin',(-44.2634,94.6262929075966,-30.));
#302914=CARTESIAN_POINT('',(-50.,94.6262929075966,-37.));
#302915=CARTESIAN_POINT('',(-6.51208132172169E-80,94.6262929075966,-37.));
#302916=CARTESIAN_POINT('Origin',(-50.,94.6262929075966,-30.));
#302917=CARTESIAN_POINT('Origin',(0.,50.6262929075966,-30.));
#302918=CARTESIAN_POINT('',(-44.2634,50.6262929075966,-37.));
#302919=CARTESIAN_POINT('Origin',(-44.2634,50.6262929075966,-30.));
#302920=CARTESIAN_POINT('',(-50.,50.6262929075966,-37.));
#302921=CARTESIAN_POINT('',(-6.51208132172169E-80,50.6262929075966,-37.));
#302922=CARTESIAN_POINT('Origin',(-50.,50.6262929075966,-30.));
#302923=CARTESIAN_POINT('Origin',(-44.2634,0.,-6.47319999999996));
#302924=CARTESIAN_POINT('',(-10.,0.,-5.73659999999998));
#302925=CARTESIAN_POINT('',(-43.5268,0.,-5.73659999999998));
#302926=CARTESIAN_POINT('',(0.,0.,-5.73659999999998));
#302927=CARTESIAN_POINT('',(-10.,0.,0.));
#302928=CARTESIAN_POINT('',(-10.,0.,-6.47319999999996));
#302929=CARTESIAN_POINT('',(-43.5268,0.,0.));
#302930=CARTESIAN_POINT('',(0.,0.,0.));
#302931=CARTESIAN_POINT('',(-43.5268,0.,0.));
#302932=CARTESIAN_POINT('Origin',(-44.2634,500.,-53.5268));
#302933=CARTESIAN_POINT('',(-43.5268,500.,-54.2634));
#302934=CARTESIAN_POINT('',(-10.,500.,-54.2634));
#302935=CARTESIAN_POINT('',(-50.,500.,-54.2634));
#302936=CARTESIAN_POINT('',(-10.,500.,-59.9999999999999));
#302937=CARTESIAN_POINT('',(-10.,500.,-53.5268));
#302938=CARTESIAN_POINT('',(-43.5268,500.,-59.9999999999999));
#302939=CARTESIAN_POINT('',(-50.,500.,-59.9999999999999));
#302940=CARTESIAN_POINT('',(-43.5268,500.,-59.9999999999999));
#302941=CARTESIAN_POINT('Origin',(-50.,500.,-54.2634));
#302942=CARTESIAN_POINT('',(-10.,0.,-54.2634));
#302943=CARTESIAN_POINT('',(-10.,500.,-54.2634));
#302944=CARTESIAN_POINT('',(-43.5268,0.,-54.2634));
#302945=CARTESIAN_POINT('',(-43.5268,500.,-54.2634));
#302946=CARTESIAN_POINT('',(-50.,0.,-54.2634));
#302947=CARTESIAN_POINT('Origin',(-50.,500.,-59.9999999999999));
#302948=CARTESIAN_POINT('',(-10.,0.,-59.9999999999999));
#302949=CARTESIAN_POINT('',(-10.,500.,-59.9999999999999));
#302950=CARTESIAN_POINT('',(-43.5268,0.,-59.9999999999999));
#302951=CARTESIAN_POINT('',(-50.,0.,-59.9999999999999));
#302952=CARTESIAN_POINT('',(-43.5268,500.,-59.9999999999999));
#302953=CARTESIAN_POINT('Origin',(0.,500.,0.));
#302954=CARTESIAN_POINT('',(-10.,500.,0.));
#302955=CARTESIAN_POINT('',(-10.,500.,0.));
#302956=CARTESIAN_POINT('',(-43.5268,500.,0.));
#302957=CARTESIAN_POINT('',(0.,500.,0.));
#302958=CARTESIAN_POINT('',(-43.5268,500.,0.));
#302959=CARTESIAN_POINT('Origin',(0.,500.,-5.73659999999998));
#302960=CARTESIAN_POINT('',(-10.,500.,-5.73659999999998));
#302961=CARTESIAN_POINT('',(-10.,500.,-5.73659999999998));
#302962=CARTESIAN_POINT('',(-43.5268,500.,-5.73659999999998));
#302963=CARTESIAN_POINT('',(-43.5268,500.,-5.73659999999998));
#302964=CARTESIAN_POINT('',(0.,500.,-5.73659999999998));
#302965=CARTESIAN_POINT('Origin',(-43.5268,500.,-53.5268));
#302966=CARTESIAN_POINT('',(-10.,500.,-53.5268));
#302967=CARTESIAN_POINT('',(-43.5268,500.,-5.73659999999998));
#302968=CARTESIAN_POINT('Origin',(-43.5268,0.,-53.5268));
#302969=CARTESIAN_POINT('',(-10.,0.,-53.5268));
#302970=CARTESIAN_POINT('',(-43.5268,0.,-54.2634));
#302971=CARTESIAN_POINT('Origin',(-50.,500.,-6.47319999999996));
#302972=CARTESIAN_POINT('',(-50.,500.,-6.47319999999996));
#302973=CARTESIAN_POINT('',(-44.2634,500.,-6.47319999999996));
#302974=CARTESIAN_POINT('',(-50.,500.,-6.47319999999996));
#302975=CARTESIAN_POINT('Origin',(-43.5268,500.,-6.47319999999996));
#302976=CARTESIAN_POINT('Origin',(-43.5268,500.,-6.47319999999996));
#302977=CARTESIAN_POINT('Origin',(-43.5268,500.,-5.73659999999998));
#302978=CARTESIAN_POINT('',(-50.,500.,-53.5268));
#302979=CARTESIAN_POINT('',(-50.,500.,0.));
#302980=CARTESIAN_POINT('',(-44.2634,500.,-53.5268));
#302981=CARTESIAN_POINT('',(-44.2634,500.,0.));
#302982=CARTESIAN_POINT('',(-44.2634,500.,-53.5268));
#302983=CARTESIAN_POINT('Origin',(-43.5268,0.,0.));
#302984=CARTESIAN_POINT('',(-50.,0.,-6.47319999999996));
#302985=CARTESIAN_POINT('Origin',(-43.5268,0.,-6.47319999999996));
#302986=CARTESIAN_POINT('',(-44.2634,0.,-6.47319999999996));
#302987=CARTESIAN_POINT('',(-44.2634,0.,-6.47319999999996));
#302988=CARTESIAN_POINT('Origin',(-43.5268,0.,-6.47319999999996));
#302989=CARTESIAN_POINT('Origin',(-43.5268,500.,-59.9999999999999));
#302990=CARTESIAN_POINT('Origin',(-43.5268,500.,-53.5268));
#302991=CARTESIAN_POINT('Origin',(-43.5268,500.,-53.5268));
#302992=CARTESIAN_POINT('Origin',(-50.,0.,-53.5268));
#302993=CARTESIAN_POINT('',(-50.,0.,-53.5268));
#302994=CARTESIAN_POINT('',(-44.2634,0.,-53.5268));
#302995=CARTESIAN_POINT('',(-50.,0.,-53.5268));
#302996=CARTESIAN_POINT('Origin',(-43.5268,0.,-53.5268));
#302997=CARTESIAN_POINT('Origin',(-43.5268,0.,-53.5268));
#302998=CARTESIAN_POINT('Origin',(-43.5268,0.,-54.2634));
#302999=CARTESIAN_POINT('',(-50.,0.,0.));
#303000=CARTESIAN_POINT('',(-44.2634,0.,0.));
#303001=CARTESIAN_POINT('Origin',(-43.5268,500.,-53.5268));
#303002=CARTESIAN_POINT('',(-50.,500.,-53.5268));
#303003=CARTESIAN_POINT('Origin',(-50.,500.,0.));
#303004=CARTESIAN_POINT('',(-50.,500.,-6.47319999999996));
#303005=CARTESIAN_POINT('Origin',(-43.5268,500.,-6.47319999999996));
#303006=CARTESIAN_POINT('Origin',(-43.5268,500.,-6.47319999999996));
#303007=CARTESIAN_POINT('',(-44.2634,500.,-6.47319999999996));
#303008=CARTESIAN_POINT('Origin',(-44.2634,500.,0.));
#303009=CARTESIAN_POINT('',(-44.2634,500.,-53.5268));
#303010=CARTESIAN_POINT('Origin',(-43.5268,500.,-53.5268));
#303011=CARTESIAN_POINT('Origin',(-10.,0.,0.));
#303012=CARTESIAN_POINT('Origin',(-10.,0.,0.));
#310597=UNCERTAINTY_MEASURE_WITH_UNIT(LENGTH_MEASURE(0.01),#310624,
'DISTANCE_ACCURACY_VALUE',
'Maximum model space distance between geometric entities at asserted c
onnectivities');
#310601=UNCERTAINTY_MEASURE_WITH_UNIT(LENGTH_MEASURE(0.01),#310624,
'DISTANCE_ACCURACY_VALUE',
'Maximum model space distance between geometric entities at asserted c
onnectivities');
#310619=(
GEOMETRIC_REPRESENTATION_CONTEXT(3)
GLOBAL_UNCERTAINTY_ASSIGNED_CONTEXT((#310597))
GLOBAL_UNIT_ASSIGNED_CONTEXT((#310624,#310626,#310627))
REPRESENTATION_CONTEXT('','3D')
);
#310623=(
GEOMETRIC_REPRESENTATION_CONTEXT(3)
GLOBAL_UNCERTAINTY_ASSIGNED_CONTEXT((#310601))
GLOBAL_UNIT_ASSIGNED_CONTEXT((#310624,#310626,#310627))
REPRESENTATION_CONTEXT('','3D')
);
#310624=(
LENGTH_UNIT()
NAMED_UNIT(*)
SI_UNIT(.MILLI.,.METRE.)
);
#310626=(
NAMED_UNIT(*)
PLANE_ANGLE_UNIT()
SI_UNIT($,.RADIAN.)
);
#310627=(
NAMED_UNIT(*)
SI_UNIT($,.STERADIAN.)
SOLID_ANGLE_UNIT()
);
#310645=SHAPE_DEFINITION_REPRESENTATION(#310804,#310910);
#310804=PRODUCT_DEFINITION_SHAPE('',$,#310932);
#310910=SHAPE_REPRESENTATION('',(#104597),#310619);
#310914=PRODUCT_DEFINITION_CONTEXT('part definition',#310979,'design');
#310932=PRODUCT_DEFINITION('Conveyor Support Leg',
'Conveyor Support Leg',#310953,#310914);
#310953=PRODUCT_DEFINITION_FORMATION('',$,#310998);
#310979=APPLICATION_CONTEXT(
'Core Data for Automotive Mechanical Design Process');
#310980=PRODUCT_CONTEXT('part definition',#310979,'mechanical');
#310998=PRODUCT('Conveyor Support Leg','Conveyor Support Leg',$,(#310980));
#311003=PRESENTATION_STYLE_ASSIGNMENT((#311010));
#311010=SURFACE_STYLE_USAGE(.BOTH.,#311017);
#311017=SURFACE_SIDE_STYLE('',(#311024));
#311024=SURFACE_STYLE_FILL_AREA(#311031);
#311031=FILL_AREA_STYLE('Opaque(97,158,199)',(#311038));
#311038=FILL_AREA_STYLE_COLOUR('Opaque(97,158,199)',#311045);
#311045=COLOUR_RGB('Opaque(97,158,199)',0.380392156862745,0.619607843137255,
0.780392156862745);
ENDSEC;
END-ISO-10303-21;
